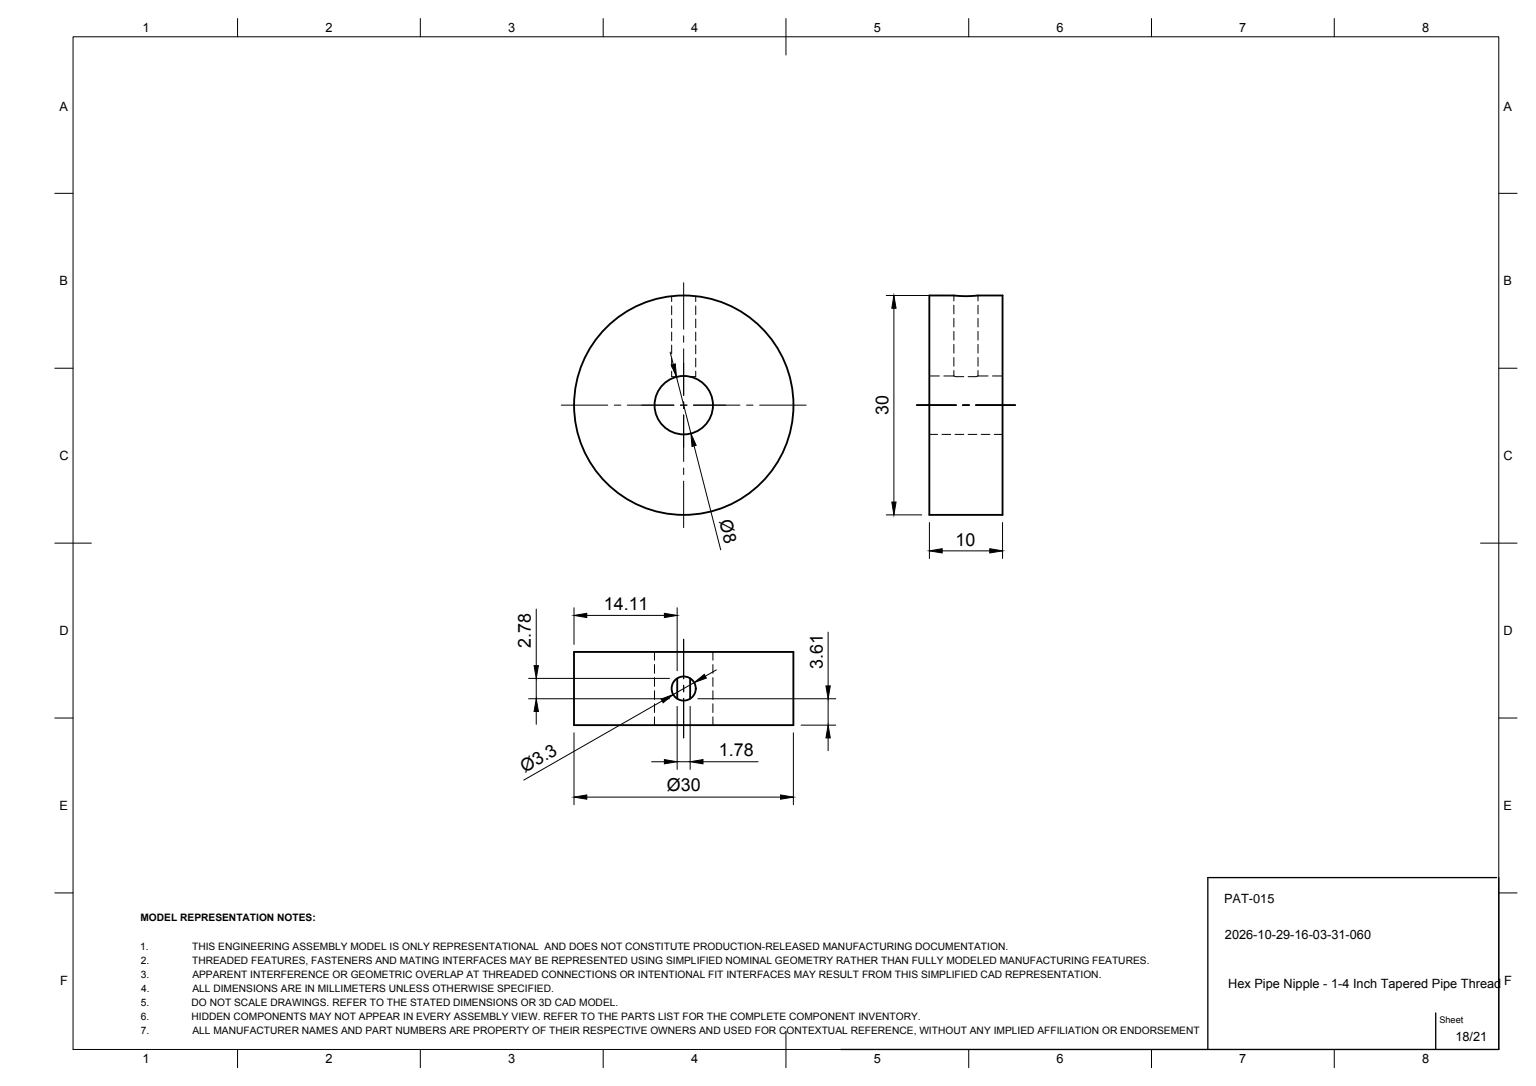
ISO-10303-21;
HEADER;
/* Generated by software containing ST-Developer
 * from STEP Tools, Inc. (www.steptools.com) 
 */

FILE_DESCRIPTION(
/* description */ ('PAT-015'),
/* implementation_level */ '2;1');

FILE_NAME(
/* name */ 'Hex Pipe Nipple - 1-4 Inch Tapered Pipe Thread.step',
/* time_stamp */ '2026-10-29T16:03:43-07:00',
/* author */ (''),
/* organization */ (''),
/* preprocessor_version */ 'ST-DEVELOPER v20.2',
/* originating_system */ 'Autodesk Translation Framework v15.17.0.0',
/* authorisation */ '');

FILE_SCHEMA (('AUTOMOTIVE_DESIGN { 1 0 10303 214 3 1 1 }'));
ENDSEC;

DATA;
#10=MECHANICAL_DESIGN_GEOMETRIC_PRESENTATION_REPRESENTATION('',(#237),#10266);
#168=CONICAL_SURFACE('',#5214,0.645,0.785398163397448);
#169=CONICAL_SURFACE('',#5217,0.645,0.785398163397448);
#189=SHAPE_REPRESENTATION_RELATIONSHIP('SRR','None',#10360,#212);
#212=ADVANCED_BREP_SHAPE_REPRESENTATION('',(#262),#10248);
#237=STYLED_ITEM('',(#10540),#262);
#262=MANIFOLD_SOLID_BREP('Body1',#4696);
#360=FACE_BOUND('',#1041,.T.);
#361=FACE_BOUND('',#1043,.T.);
#362=FACE_BOUND('',#1052,.T.);
#363=FACE_BOUND('',#1057,.T.);
#477=PLANE('',#5199);
#478=PLANE('',#5201);
#479=PLANE('',#5203);
#480=PLANE('',#5204);
#481=PLANE('',#5205);
#482=PLANE('',#5206);
#483=PLANE('',#5207);
#484=PLANE('',#5208);
#485=PLANE('',#5211);
#486=PLANE('',#5219);
#689=FACE_OUTER_BOUND('',#1040,.T.);
#690=FACE_OUTER_BOUND('',#1042,.T.);
#691=FACE_OUTER_BOUND('',#1044,.T.);
#692=FACE_OUTER_BOUND('',#1045,.T.);
#693=FACE_OUTER_BOUND('',#1046,.T.);
#694=FACE_OUTER_BOUND('',#1047,.T.);
#695=FACE_OUTER_BOUND('',#1048,.T.);
#696=FACE_OUTER_BOUND('',#1049,.T.);
#697=FACE_OUTER_BOUND('',#1050,.T.);
#698=FACE_OUTER_BOUND('',#1051,.T.);
#699=FACE_OUTER_BOUND('',#1053,.T.);
#700=FACE_OUTER_BOUND('',#1054,.T.);
#701=FACE_OUTER_BOUND('',#1055,.T.);
#702=FACE_OUTER_BOUND('',#1056,.T.);
#703=FACE_OUTER_BOUND('',#1058,.T.);
#1040=EDGE_LOOP('',(#3643,#3644,#3645,#3646,#3647,#3648));
#1041=EDGE_LOOP('',(#3649));
#1042=EDGE_LOOP('',(#3650,#3651,#3652,#3653,#3654,#3655));
#1043=EDGE_LOOP('',(#3656));
#1044=EDGE_LOOP('',(#3657,#3658,#3659,#3660));
#1045=EDGE_LOOP('',(#3661,#3662,#3663,#3664));
#1046=EDGE_LOOP('',(#3665,#3666,#3667,#3668));
#1047=EDGE_LOOP('',(#3669,#3670,#3671,#3672));
#1048=EDGE_LOOP('',(#3673,#3674,#3675,#3676));
#1049=EDGE_LOOP('',(#3677,#3678,#3679,#3680));
#1050=EDGE_LOOP('',(#3681,#3682,#3683,#3684));
#1051=EDGE_LOOP('',(#3685));
#1052=EDGE_LOOP('',(#3686));
#1053=EDGE_LOOP('',(#3687,#3688,#3689,#3690));
#1054=EDGE_LOOP('',(#3691,#3692,#3693,#3694));
#1055=EDGE_LOOP('',(#3695,#3696,#3697,#3698));
#1056=EDGE_LOOP('',(#3699));
#1057=EDGE_LOOP('',(#3700));
#1058=EDGE_LOOP('',(#3701,#3702,#3703,#3704));
#1436=LINE('',#8614,#1716);
#1437=LINE('',#8616,#1717);
#1438=LINE('',#8618,#1718);
#1439=LINE('',#8620,#1719);
#1440=LINE('',#8622,#1720);
#1441=LINE('',#8623,#1721);
#1442=LINE('',#8629,#1722);
#1443=LINE('',#8631,#1723);
#1444=LINE('',#8633,#1724);
#1445=LINE('',#8635,#1725);
#1446=LINE('',#8637,#1726);
#1447=LINE('',#8638,#1727);
#1448=LINE('',#8642,#1728);
#1449=LINE('',#8643,#1729);
#1450=LINE('',#8645,#1730);
#1451=LINE('',#8647,#1731);
#1452=LINE('',#8649,#1732);
#1453=LINE('',#8651,#1733);
#1454=LINE('',#8655,#1734);
#1455=LINE('',#8663,#1735);
#1456=LINE('',#8667,#1736);
#1457=LINE('',#8671,#1737);
#1458=LINE('',#8676,#1738);
#1716=VECTOR('',#6129,1.);
#1717=VECTOR('',#6130,1.);
#1718=VECTOR('',#6131,1.);
#1719=VECTOR('',#6132,1.);
#1720=VECTOR('',#6133,1.);
#1721=VECTOR('',#6134,1.);
#1722=VECTOR('',#6139,1.);
#1723=VECTOR('',#6140,1.);
#1724=VECTOR('',#6141,1.);
#1725=VECTOR('',#6142,1.);
#1726=VECTOR('',#6143,1.);
#1727=VECTOR('',#6144,1.);
#1728=VECTOR('',#6149,1.);
#1729=VECTOR('',#6150,1.);
#1730=VECTOR('',#6153,1.);
#1731=VECTOR('',#6156,1.);
#1732=VECTOR('',#6159,1.);
#1733=VECTOR('',#6162,1.);
#1734=VECTOR('',#6167,0.685);
#1735=VECTOR('',#6178,0.645);
#1736=VECTOR('',#6183,0.685);
#1737=VECTOR('',#6188,0.645);
#1738=VECTOR('',#6195,0.46);
#1973=CIRCLE('',#5200,0.685);
#1974=CIRCLE('',#5202,0.685);
#1975=CIRCLE('',#5210,0.685);
#1976=CIRCLE('',#5212,0.605);
#1977=CIRCLE('',#5213,0.46);
#1978=CIRCLE('',#5216,0.685);
#1979=CIRCLE('',#5218,0.605);
#1980=CIRCLE('',#5220,0.46);
#2295=VERTEX_POINT('',#8612);
#2296=VERTEX_POINT('',#8613);
#2297=VERTEX_POINT('',#8615);
#2298=VERTEX_POINT('',#8617);
#2299=VERTEX_POINT('',#8619);
#2300=VERTEX_POINT('',#8621);
#2301=VERTEX_POINT('',#8624);
#2302=VERTEX_POINT('',#8627);
#2303=VERTEX_POINT('',#8628);
#2304=VERTEX_POINT('',#8630);
#2305=VERTEX_POINT('',#8632);
#2306=VERTEX_POINT('',#8634);
#2307=VERTEX_POINT('',#8636);
#2308=VERTEX_POINT('',#8639);
#2309=VERTEX_POINT('',#8654);
#2310=VERTEX_POINT('',#8658);
#2311=VERTEX_POINT('',#8660);
#2312=VERTEX_POINT('',#8665);
#2313=VERTEX_POINT('',#8669);
#2314=VERTEX_POINT('',#8673);
#2777=EDGE_CURVE('',#2295,#2296,#1436,.T.);
#2778=EDGE_CURVE('',#2296,#2297,#1437,.T.);
#2779=EDGE_CURVE('',#2297,#2298,#1438,.T.);
#2780=EDGE_CURVE('',#2298,#2299,#1439,.T.);
#2781=EDGE_CURVE('',#2299,#2300,#1440,.T.);
#2782=EDGE_CURVE('',#2300,#2295,#1441,.T.);
#2783=EDGE_CURVE('',#2301,#2301,#1973,.T.);
#2784=EDGE_CURVE('',#2302,#2303,#1442,.T.);
#2785=EDGE_CURVE('',#2303,#2304,#1443,.T.);
#2786=EDGE_CURVE('',#2304,#2305,#1444,.T.);
#2787=EDGE_CURVE('',#2305,#2306,#1445,.T.);
#2788=EDGE_CURVE('',#2306,#2307,#1446,.T.);
#2789=EDGE_CURVE('',#2307,#2302,#1447,.T.);
#2790=EDGE_CURVE('',#2308,#2308,#1974,.T.);
#2791=EDGE_CURVE('',#2302,#2296,#1448,.T.);
#2792=EDGE_CURVE('',#2297,#2307,#1449,.T.);
#2793=EDGE_CURVE('',#2298,#2306,#1450,.T.);
#2794=EDGE_CURVE('',#2299,#2305,#1451,.T.);
#2795=EDGE_CURVE('',#2300,#2304,#1452,.T.);
#2796=EDGE_CURVE('',#2295,#2303,#1453,.T.);
#2797=EDGE_CURVE('',#2308,#2309,#1454,.T.);
#2798=EDGE_CURVE('',#2309,#2309,#1975,.T.);
#2799=EDGE_CURVE('',#2310,#2310,#1976,.T.);
#2800=EDGE_CURVE('',#2311,#2311,#1977,.T.);
#2801=EDGE_CURVE('',#2309,#2310,#1455,.T.);
#2802=EDGE_CURVE('',#2312,#2312,#1978,.T.);
#2803=EDGE_CURVE('',#2312,#2301,#1456,.T.);
#2804=EDGE_CURVE('',#2313,#2313,#1979,.T.);
#2805=EDGE_CURVE('',#2313,#2312,#1457,.T.);
#2806=EDGE_CURVE('',#2314,#2314,#1980,.T.);
#2807=EDGE_CURVE('',#2314,#2311,#1458,.T.);
#3643=ORIENTED_EDGE('',*,*,#2777,.T.);
#3644=ORIENTED_EDGE('',*,*,#2778,.T.);
#3645=ORIENTED_EDGE('',*,*,#2779,.T.);
#3646=ORIENTED_EDGE('',*,*,#2780,.T.);
#3647=ORIENTED_EDGE('',*,*,#2781,.T.);
#3648=ORIENTED_EDGE('',*,*,#2782,.T.);
#3649=ORIENTED_EDGE('',*,*,#2783,.F.);
#3650=ORIENTED_EDGE('',*,*,#2784,.T.);
#3651=ORIENTED_EDGE('',*,*,#2785,.T.);
#3652=ORIENTED_EDGE('',*,*,#2786,.T.);
#3653=ORIENTED_EDGE('',*,*,#2787,.T.);
#3654=ORIENTED_EDGE('',*,*,#2788,.T.);
#3655=ORIENTED_EDGE('',*,*,#2789,.T.);
#3656=ORIENTED_EDGE('',*,*,#2790,.F.);
#3657=ORIENTED_EDGE('',*,*,#2791,.F.);
#3658=ORIENTED_EDGE('',*,*,#2789,.F.);
#3659=ORIENTED_EDGE('',*,*,#2792,.F.);
#3660=ORIENTED_EDGE('',*,*,#2778,.F.);
#3661=ORIENTED_EDGE('',*,*,#2792,.T.);
#3662=ORIENTED_EDGE('',*,*,#2788,.F.);
#3663=ORIENTED_EDGE('',*,*,#2793,.F.);
#3664=ORIENTED_EDGE('',*,*,#2779,.F.);
#3665=ORIENTED_EDGE('',*,*,#2793,.T.);
#3666=ORIENTED_EDGE('',*,*,#2787,.F.);
#3667=ORIENTED_EDGE('',*,*,#2794,.F.);
#3668=ORIENTED_EDGE('',*,*,#2780,.F.);
#3669=ORIENTED_EDGE('',*,*,#2794,.T.);
#3670=ORIENTED_EDGE('',*,*,#2786,.F.);
#3671=ORIENTED_EDGE('',*,*,#2795,.F.);
#3672=ORIENTED_EDGE('',*,*,#2781,.F.);
#3673=ORIENTED_EDGE('',*,*,#2795,.T.);
#3674=ORIENTED_EDGE('',*,*,#2785,.F.);
#3675=ORIENTED_EDGE('',*,*,#2796,.F.);
#3676=ORIENTED_EDGE('',*,*,#2782,.F.);
#3677=ORIENTED_EDGE('',*,*,#2796,.T.);
#3678=ORIENTED_EDGE('',*,*,#2784,.F.);
#3679=ORIENTED_EDGE('',*,*,#2791,.T.);
#3680=ORIENTED_EDGE('',*,*,#2777,.F.);
#3681=ORIENTED_EDGE('',*,*,#2790,.T.);
#3682=ORIENTED_EDGE('',*,*,#2797,.T.);
#3683=ORIENTED_EDGE('',*,*,#2798,.T.);
#3684=ORIENTED_EDGE('',*,*,#2797,.F.);
#3685=ORIENTED_EDGE('',*,*,#2799,.F.);
#3686=ORIENTED_EDGE('',*,*,#2800,.T.);
#3687=ORIENTED_EDGE('',*,*,#2798,.F.);
#3688=ORIENTED_EDGE('',*,*,#2801,.T.);
#3689=ORIENTED_EDGE('',*,*,#2799,.T.);
#3690=ORIENTED_EDGE('',*,*,#2801,.F.);
#3691=ORIENTED_EDGE('',*,*,#2802,.F.);
#3692=ORIENTED_EDGE('',*,*,#2803,.T.);
#3693=ORIENTED_EDGE('',*,*,#2783,.T.);
#3694=ORIENTED_EDGE('',*,*,#2803,.F.);
#3695=ORIENTED_EDGE('',*,*,#2804,.F.);
#3696=ORIENTED_EDGE('',*,*,#2805,.T.);
#3697=ORIENTED_EDGE('',*,*,#2802,.T.);
#3698=ORIENTED_EDGE('',*,*,#2805,.F.);
#3699=ORIENTED_EDGE('',*,*,#2804,.T.);
#3700=ORIENTED_EDGE('',*,*,#2806,.F.);
#3701=ORIENTED_EDGE('',*,*,#2806,.T.);
#3702=ORIENTED_EDGE('',*,*,#2807,.T.);
#3703=ORIENTED_EDGE('',*,*,#2800,.F.);
#3704=ORIENTED_EDGE('',*,*,#2807,.F.);
#4351=CYLINDRICAL_SURFACE('',#5209,0.685);
#4352=CYLINDRICAL_SURFACE('',#5215,0.685);
#4353=CYLINDRICAL_SURFACE('',#5221,0.46);
#4524=ADVANCED_FACE('',(#689,#360),#477,.F.);
#4525=ADVANCED_FACE('',(#690,#361),#478,.T.);
#4526=ADVANCED_FACE('',(#691),#479,.T.);
#4527=ADVANCED_FACE('',(#692),#480,.T.);
#4528=ADVANCED_FACE('',(#693),#481,.T.);
#4529=ADVANCED_FACE('',(#694),#482,.T.);
#4530=ADVANCED_FACE('',(#695),#483,.T.);
#4531=ADVANCED_FACE('',(#696),#484,.T.);
#4532=ADVANCED_FACE('',(#697),#4351,.T.);
#4533=ADVANCED_FACE('',(#698,#362),#485,.T.);
#4534=ADVANCED_FACE('',(#699),#168,.T.);
#4535=ADVANCED_FACE('',(#700),#4352,.T.);
#4536=ADVANCED_FACE('',(#701),#169,.T.);
#4537=ADVANCED_FACE('',(#702,#363),#486,.T.);
#4538=ADVANCED_FACE('',(#703),#4353,.F.);
#4696=CLOSED_SHELL('',(#4524,#4525,#4526,#4527,#4528,#4529,#4530,#4531,
#4532,#4533,#4534,#4535,#4536,#4537,#4538));
#5198=AXIS2_PLACEMENT_3D('',#8610,#6125,#6126);
#5199=AXIS2_PLACEMENT_3D('',#8611,#6127,#6128);
#5200=AXIS2_PLACEMENT_3D('',#8625,#6135,#6136);
#5201=AXIS2_PLACEMENT_3D('',#8626,#6137,#6138);
#5202=AXIS2_PLACEMENT_3D('',#8640,#6145,#6146);
#5203=AXIS2_PLACEMENT_3D('',#8641,#6147,#6148);
#5204=AXIS2_PLACEMENT_3D('',#8644,#6151,#6152);
#5205=AXIS2_PLACEMENT_3D('',#8646,#6154,#6155);
#5206=AXIS2_PLACEMENT_3D('',#8648,#6157,#6158);
#5207=AXIS2_PLACEMENT_3D('',#8650,#6160,#6161);
#5208=AXIS2_PLACEMENT_3D('',#8652,#6163,#6164);
#5209=AXIS2_PLACEMENT_3D('',#8653,#6165,#6166);
#5210=AXIS2_PLACEMENT_3D('',#8656,#6168,#6169);
#5211=AXIS2_PLACEMENT_3D('',#8657,#6170,#6171);
#5212=AXIS2_PLACEMENT_3D('',#8659,#6172,#6173);
#5213=AXIS2_PLACEMENT_3D('',#8661,#6174,#6175);
#5214=AXIS2_PLACEMENT_3D('',#8662,#6176,#6177);
#5215=AXIS2_PLACEMENT_3D('',#8664,#6179,#6180);
#5216=AXIS2_PLACEMENT_3D('',#8666,#6181,#6182);
#5217=AXIS2_PLACEMENT_3D('',#8668,#6184,#6185);
#5218=AXIS2_PLACEMENT_3D('',#8670,#6186,#6187);
#5219=AXIS2_PLACEMENT_3D('',#8672,#6189,#6190);
#5220=AXIS2_PLACEMENT_3D('',#8674,#6191,#6192);
#5221=AXIS2_PLACEMENT_3D('',#8675,#6193,#6194);
#6125=DIRECTION('axis',(0.,0.,1.));
#6126=DIRECTION('refdir',(1.,0.,0.));
#6127=DIRECTION('center_axis',(0.,1.,0.));
#6128=DIRECTION('ref_axis',(1.,0.,0.));
#6129=DIRECTION('',(-0.5,0.,0.866025403784439));
#6130=DIRECTION('',(-1.,0.,-3.29650746237182E-16));
#6131=DIRECTION('',(-0.5,0.,-0.866025403784439));
#6132=DIRECTION('',(0.5,0.,-0.866025403784438));
#6133=DIRECTION('',(1.,0.,0.));
#6134=DIRECTION('',(0.5,0.,0.866025403784439));
#6135=DIRECTION('center_axis',(0.,-1.,0.));
#6136=DIRECTION('ref_axis',(1.,0.,0.));
#6137=DIRECTION('center_axis',(0.,1.,0.));
#6138=DIRECTION('ref_axis',(1.,0.,0.));
#6139=DIRECTION('',(0.5,0.,-0.866025403784439));
#6140=DIRECTION('',(-0.5,0.,-0.866025403784439));
#6141=DIRECTION('',(-1.,0.,0.));
#6142=DIRECTION('',(-0.5,0.,0.866025403784438));
#6143=DIRECTION('',(0.5,0.,0.866025403784439));
#6144=DIRECTION('',(1.,0.,3.29650746237182E-16));
#6145=DIRECTION('center_axis',(0.,1.,0.));
#6146=DIRECTION('ref_axis',(1.,0.,0.));
#6147=DIRECTION('center_axis',(-3.29650746237182E-16,0.,1.));
#6148=DIRECTION('ref_axis',(1.,0.,3.29650746237182E-16));
#6149=DIRECTION('',(0.,-1.,0.));
#6150=DIRECTION('',(0.,1.,0.));
#6151=DIRECTION('center_axis',(-0.866025403784439,0.,0.5));
#6152=DIRECTION('ref_axis',(0.5,0.,0.866025403784439));
#6153=DIRECTION('',(0.,1.,0.));
#6154=DIRECTION('center_axis',(-0.866025403784439,0.,-0.5));
#6155=DIRECTION('ref_axis',(-0.5,0.,0.866025403784439));
#6156=DIRECTION('',(0.,1.,0.));
#6157=DIRECTION('center_axis',(0.,0.,-1.));
#6158=DIRECTION('ref_axis',(-1.,0.,0.));
#6159=DIRECTION('',(0.,1.,0.));
#6160=DIRECTION('center_axis',(0.866025403784439,0.,-0.5));
#6161=DIRECTION('ref_axis',(-0.5,0.,-0.866025403784439));
#6162=DIRECTION('',(0.,1.,0.));
#6163=DIRECTION('center_axis',(0.866025403784439,0.,0.5));
#6164=DIRECTION('ref_axis',(0.5,0.,-0.866025403784439));
#6165=DIRECTION('center_axis',(0.,-1.,0.));
#6166=DIRECTION('ref_axis',(1.,0.,0.));
#6167=DIRECTION('',(0.,1.,0.));
#6168=DIRECTION('center_axis',(0.,-1.,0.));
#6169=DIRECTION('ref_axis',(1.,0.,0.));
#6170=DIRECTION('center_axis',(0.,1.,0.));
#6171=DIRECTION('ref_axis',(0.,0.,1.));
#6172=DIRECTION('center_axis',(0.,-1.,0.));
#6173=DIRECTION('ref_axis',(1.,0.,0.));
#6174=DIRECTION('center_axis',(0.,-1.,0.));
#6175=DIRECTION('ref_axis',(1.,0.,0.));
#6176=DIRECTION('center_axis',(0.,-1.,0.));
#6177=DIRECTION('ref_axis',(1.,0.,0.));
#6178=DIRECTION('',(0.707106781186547,0.707106781186548,8.65956056235493E-17));
#6179=DIRECTION('center_axis',(0.,-1.,0.));
#6180=DIRECTION('ref_axis',(1.,0.,0.));
#6181=DIRECTION('center_axis',(0.,-1.,0.));
#6182=DIRECTION('ref_axis',(1.,0.,0.));
#6183=DIRECTION('',(0.,1.,0.));
#6184=DIRECTION('center_axis',(0.,1.,0.));
#6185=DIRECTION('ref_axis',(1.,0.,0.));
#6186=DIRECTION('center_axis',(0.,-1.,0.));
#6187=DIRECTION('ref_axis',(1.,0.,0.));
#6188=DIRECTION('',(-0.707106781186547,0.707106781186548,-8.65956056235493E-17));
#6189=DIRECTION('center_axis',(0.,-1.,0.));
#6190=DIRECTION('ref_axis',(0.,0.,-1.));
#6191=DIRECTION('center_axis',(0.,-1.,0.));
#6192=DIRECTION('ref_axis',(1.,0.,0.));
#6193=DIRECTION('center_axis',(0.,-1.,0.));
#6194=DIRECTION('ref_axis',(1.,0.,0.));
#6195=DIRECTION('',(0.,1.,0.));
#8610=CARTESIAN_POINT('',(0.,0.,0.));
#8611=CARTESIAN_POINT('Origin',(0.,-0.4,0.));
#8612=CARTESIAN_POINT('',(1.01036297108185,-0.4,0.));
#8613=CARTESIAN_POINT('',(0.505181485540923,-0.4,0.875));
#8614=CARTESIAN_POINT('',(0.505181485540923,-0.4,0.875));
#8615=CARTESIAN_POINT('',(-0.505181485540923,-0.4,0.875));
#8616=CARTESIAN_POINT('',(-0.505181485540923,-0.4,0.875));
#8617=CARTESIAN_POINT('',(-1.01036297108185,-0.4,-1.23733777851239E-16));
#8618=CARTESIAN_POINT('',(-1.01036297108185,-0.4,-1.23733777851239E-16));
#8619=CARTESIAN_POINT('',(-0.505181485540922,-0.4,-0.875));
#8620=CARTESIAN_POINT('',(-0.505181485540922,-0.4,-0.875));
#8621=CARTESIAN_POINT('',(0.505181485540923,-0.4,-0.875));
#8622=CARTESIAN_POINT('',(0.505181485540923,-0.4,-0.875));
#8623=CARTESIAN_POINT('',(1.01036297108185,-0.4,0.));
#8624=CARTESIAN_POINT('',(-0.685,-0.4,-8.38883057415937E-17));
#8625=CARTESIAN_POINT('Origin',(0.,-0.4,0.));
#8626=CARTESIAN_POINT('Origin',(0.,0.4,0.));
#8627=CARTESIAN_POINT('',(0.505181485540923,0.4,0.875));
#8628=CARTESIAN_POINT('',(1.01036297108185,0.4,0.));
#8629=CARTESIAN_POINT('',(0.505181485540923,0.4,0.875));
#8630=CARTESIAN_POINT('',(0.505181485540923,0.4,-0.875));
#8631=CARTESIAN_POINT('',(1.01036297108185,0.4,0.));
#8632=CARTESIAN_POINT('',(-0.505181485540922,0.4,-0.875));
#8633=CARTESIAN_POINT('',(0.505181485540923,0.4,-0.875));
#8634=CARTESIAN_POINT('',(-1.01036297108185,0.4,-1.23733777851239E-16));
#8635=CARTESIAN_POINT('',(-0.505181485540922,0.4,-0.875));
#8636=CARTESIAN_POINT('',(-0.505181485540923,0.4,0.875));
#8637=CARTESIAN_POINT('',(-1.01036297108185,0.4,-1.23733777851239E-16));
#8638=CARTESIAN_POINT('',(-0.505181485540923,0.4,0.875));
#8639=CARTESIAN_POINT('',(-0.685,0.4,8.38883057415937E-17));
#8640=CARTESIAN_POINT('Origin',(0.,0.4,0.));
#8641=CARTESIAN_POINT('Origin',(-0.505181485540923,0.,0.875));
#8642=CARTESIAN_POINT('',(0.505181485540923,0.,0.875));
#8643=CARTESIAN_POINT('',(-0.505181485540923,0.,0.875));
#8644=CARTESIAN_POINT('Origin',(-1.01036297108185,0.,-1.23733777851239E-16));
#8645=CARTESIAN_POINT('',(-1.01036297108185,0.,-1.23733777851239E-16));
#8646=CARTESIAN_POINT('Origin',(-0.505181485540922,0.,-0.875));
#8647=CARTESIAN_POINT('',(-0.505181485540922,0.,-0.875));
#8648=CARTESIAN_POINT('Origin',(0.505181485540923,0.,-0.875));
#8649=CARTESIAN_POINT('',(0.505181485540923,0.,-0.875));
#8650=CARTESIAN_POINT('Origin',(1.01036297108185,0.,0.));
#8651=CARTESIAN_POINT('',(1.01036297108185,0.,0.));
#8652=CARTESIAN_POINT('Origin',(0.505181485540923,0.,0.875));
#8653=CARTESIAN_POINT('Origin',(0.,0.,0.));
#8654=CARTESIAN_POINT('',(-0.685,1.82,-8.38883057415937E-17));
#8655=CARTESIAN_POINT('',(-0.685,0.,-8.38883057415937E-17));
#8656=CARTESIAN_POINT('Origin',(0.,1.82,0.));
#8657=CARTESIAN_POINT('Origin',(0.605,1.9,0.));
#8658=CARTESIAN_POINT('',(-0.605,1.9,-7.40911313484149E-17));
#8659=CARTESIAN_POINT('Origin',(0.,1.9,0.));
#8660=CARTESIAN_POINT('',(-0.46,1.9,-5.63337527607782E-17));
#8661=CARTESIAN_POINT('Origin',(0.,1.9,0.));
#8662=CARTESIAN_POINT('Origin',(0.,1.86,0.));
#8663=CARTESIAN_POINT('',(-0.645,1.86,-7.89897185450043E-17));
#8664=CARTESIAN_POINT('Origin',(0.,0.,0.));
#8665=CARTESIAN_POINT('',(-0.685,-1.82,-8.38883057415937E-17));
#8666=CARTESIAN_POINT('Origin',(0.,-1.82,0.));
#8667=CARTESIAN_POINT('',(-0.685,0.,-8.38883057415937E-17));
#8668=CARTESIAN_POINT('Origin',(0.,-1.86,0.));
#8669=CARTESIAN_POINT('',(-0.605,-1.9,-7.40911313484149E-17));
#8670=CARTESIAN_POINT('Origin',(0.,-1.9,0.));
#8671=CARTESIAN_POINT('',(-0.645,-1.86,-7.89897185450043E-17));
#8672=CARTESIAN_POINT('Origin',(0.46,-1.9,0.));
#8673=CARTESIAN_POINT('',(-0.46,-1.9,-5.63337527607782E-17));
#8674=CARTESIAN_POINT('Origin',(0.,-1.9,0.));
#8675=CARTESIAN_POINT('Origin',(0.,0.,0.));
#8676=CARTESIAN_POINT('',(-0.46,0.,-5.63337527607782E-17));
#10223=UNCERTAINTY_MEASURE_WITH_UNIT(LENGTH_MEASURE(0.001),#10267,
'DISTANCE_ACCURACY_VALUE',
'Maximum model space distance between geometric entities at asserted c
onnectivities');
#10241=UNCERTAINTY_MEASURE_WITH_UNIT(LENGTH_MEASURE(0.001),#10267,
'DISTANCE_ACCURACY_VALUE',
'Maximum model space distance between geometric entities at asserted c
onnectivities');
#10248=(
GEOMETRIC_REPRESENTATION_CONTEXT(3)
GLOBAL_UNCERTAINTY_ASSIGNED_CONTEXT((#10223))
GLOBAL_UNIT_ASSIGNED_CONTEXT((#10267,#10269,#10270))
REPRESENTATION_CONTEXT('','3D')
);
#10266=(
GEOMETRIC_REPRESENTATION_CONTEXT(3)
GLOBAL_UNCERTAINTY_ASSIGNED_CONTEXT((#10241))
GLOBAL_UNIT_ASSIGNED_CONTEXT((#10267,#10269,#10270))
REPRESENTATION_CONTEXT('','3D')
);
#10267=(
LENGTH_UNIT()
NAMED_UNIT(*)
SI_UNIT(.CENTI.,.METRE.)
);
#10269=(
NAMED_UNIT(*)
PLANE_ANGLE_UNIT()
SI_UNIT($,.RADIAN.)
);
#10270=(
NAMED_UNIT(*)
SI_UNIT($,.STERADIAN.)
SOLID_ANGLE_UNIT()
);
#10277=SHAPE_DEFINITION_REPRESENTATION(#10301,#10360);
#10301=PRODUCT_DEFINITION_SHAPE('',$,#10385);
#10360=SHAPE_REPRESENTATION('',(#5198),#10248);
#10378=PRODUCT_DEFINITION_CONTEXT('part definition',#10452,'design');
#10385=PRODUCT_DEFINITION('Hex Pipe Nipple - 1-4 Inch Tapered Pipe Thread',
'Hex Pipe Nipple - 1-4 Inch Tapered Pipe Thread',#10409,#10378);
#10409=PRODUCT_DEFINITION_FORMATION('',$,#10460);
#10452=APPLICATION_CONTEXT(
'Core Data for Automotive Mechanical Design Process');
#10453=PRODUCT_CONTEXT('part definition',#10452,'mechanical');
#10460=PRODUCT('Hex Pipe Nipple - 1-4 Inch Tapered Pipe Thread',
'Hex Pipe Nipple - 1-4 Inch Tapered Pipe Thread',
'Hex Pipe Nipple - 1-4 Inch Tapered Pipe Thread',(#10453));
#10534=COLOUR_RGB('Sky Blue',0.24,0.69,0.87);
#10535=FILL_AREA_STYLE_COLOUR('',#10534);
#10536=FILL_AREA_STYLE('',(#10535));
#10537=SURFACE_STYLE_FILL_AREA(#10536);
#10538=SURFACE_SIDE_STYLE('',(#10537));
#10539=SURFACE_STYLE_USAGE(.BOTH.,#10538);
#10540=PRESENTATION_STYLE_ASSIGNMENT((#10539));
ENDSEC;
END-ISO-10303-21;
